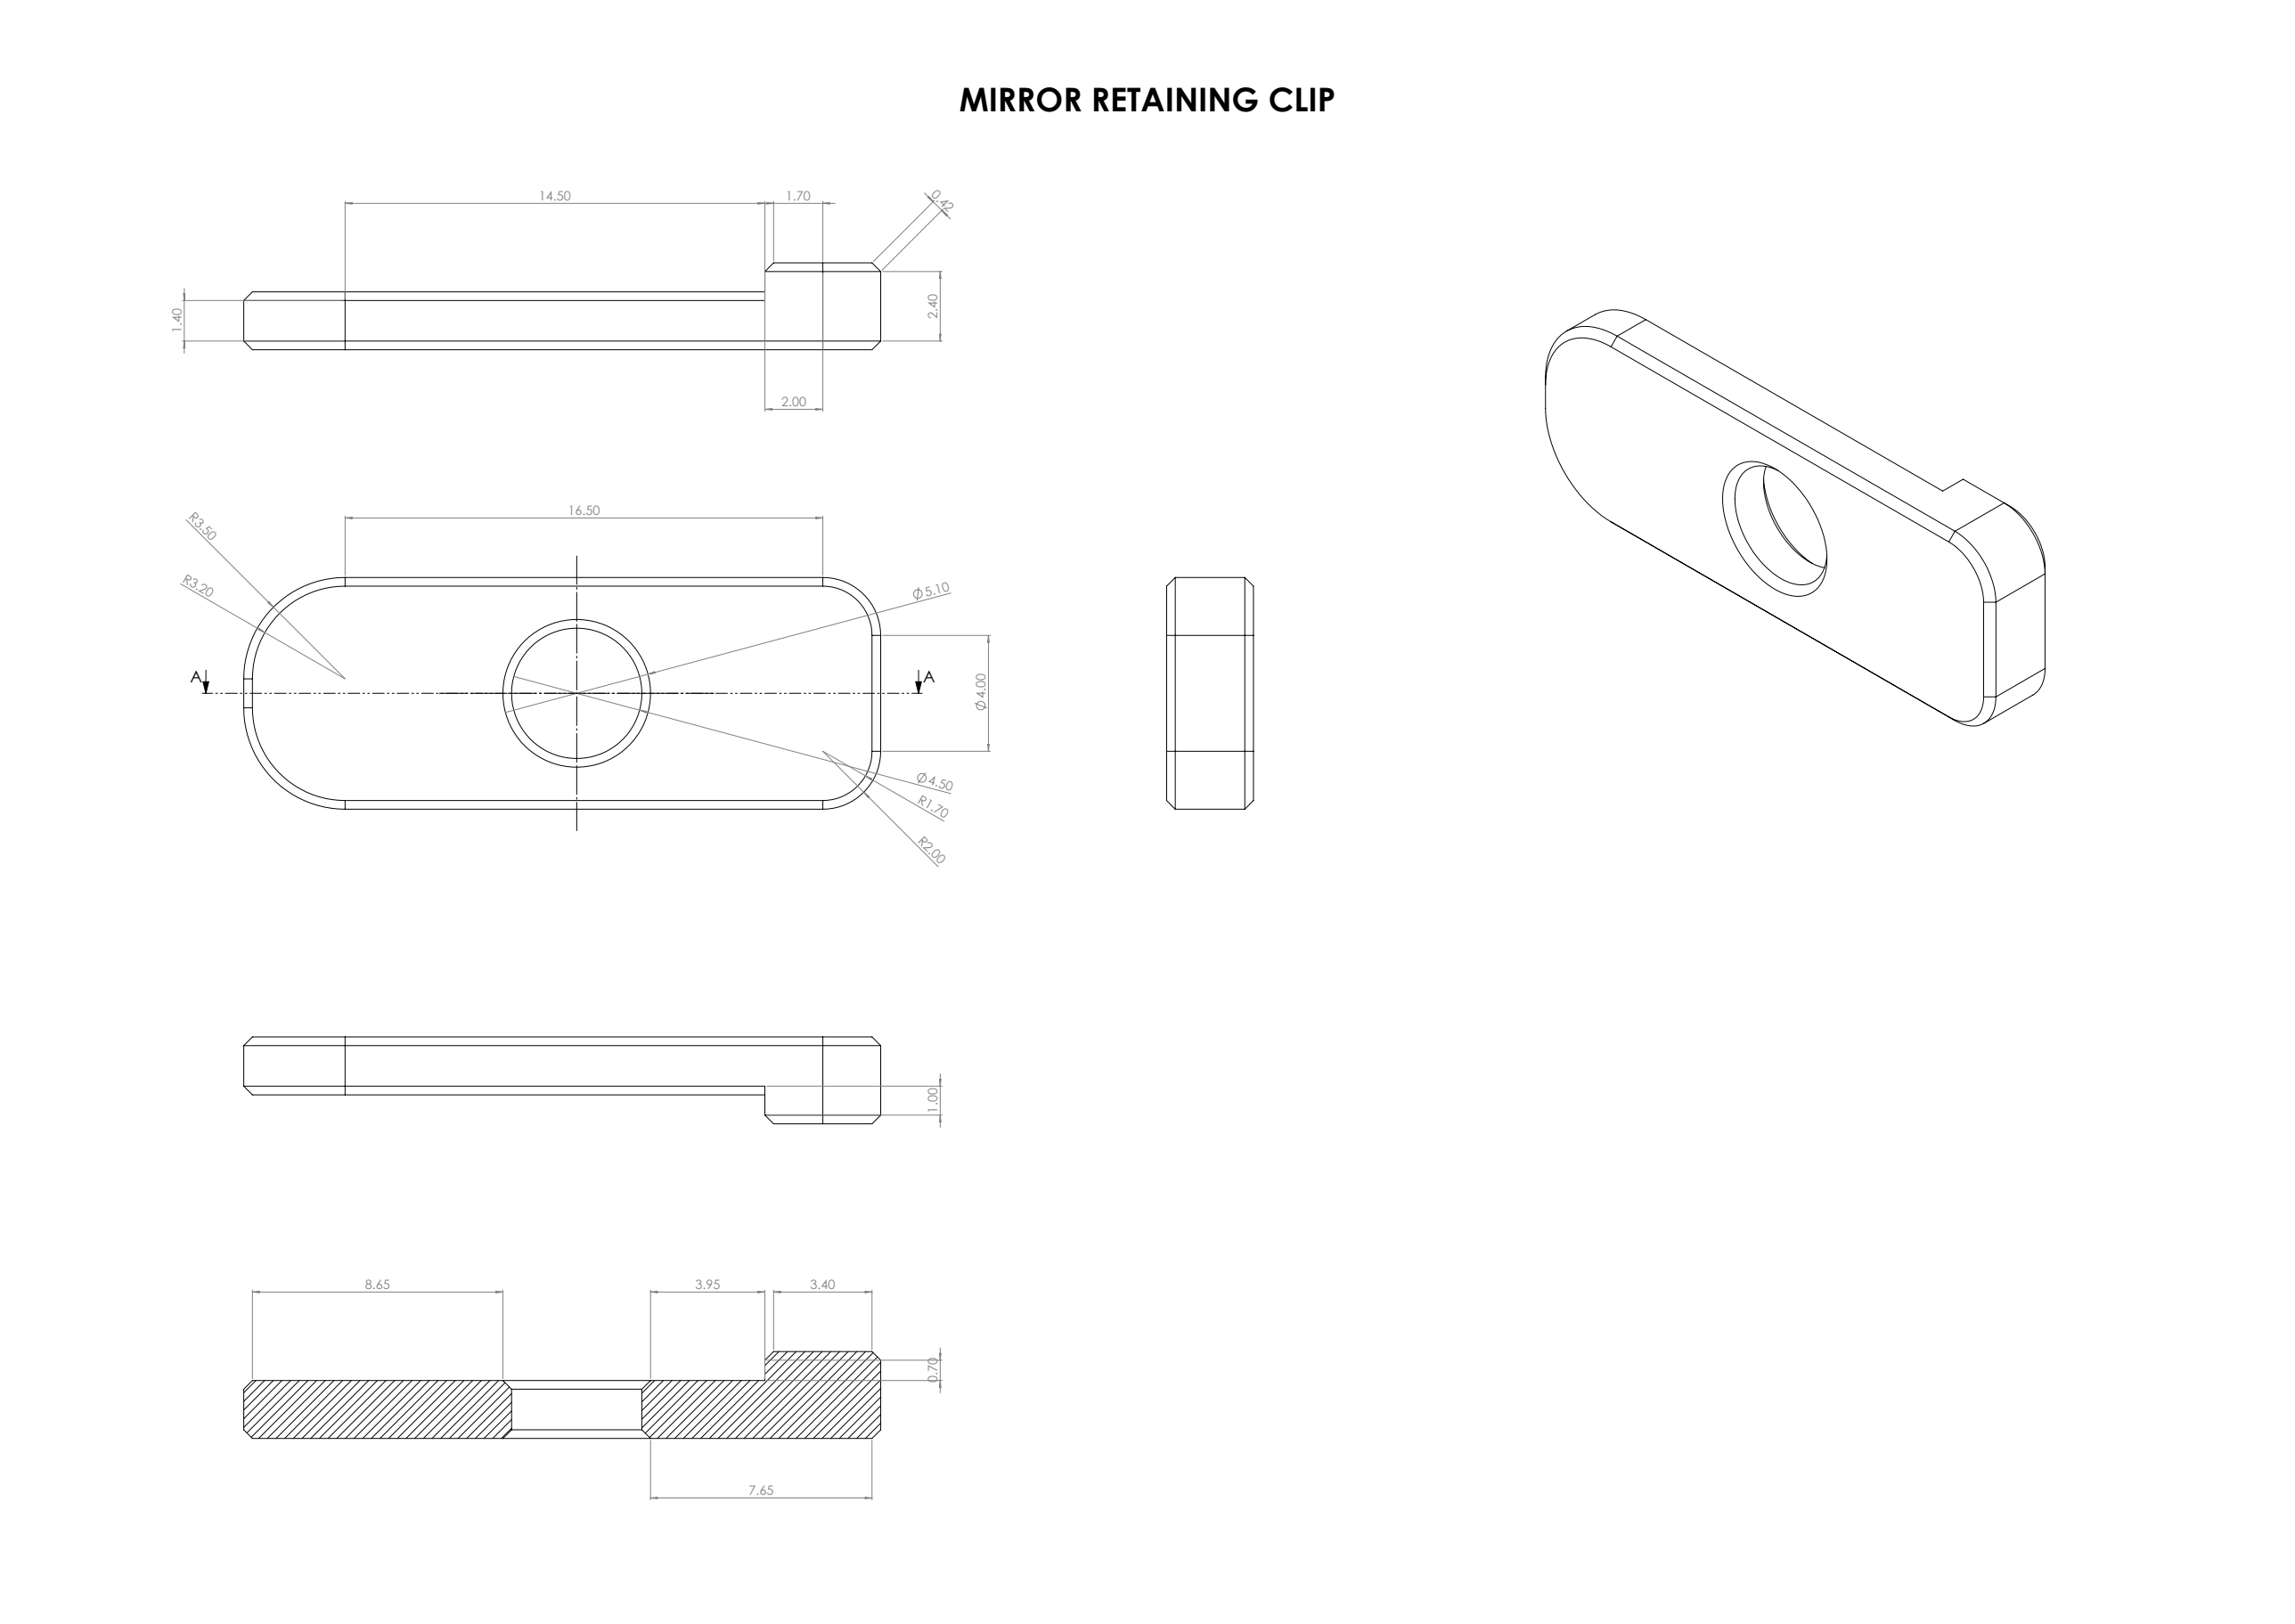
ISO-10303-21;
HEADER;
/* Generated by software containing ST-Developer
 * from STEP Tools, Inc. (www.steptools.com) 
 */

FILE_DESCRIPTION(
/* description */ (''),
/* implementation_level */ '2;1');

FILE_NAME(
/* name */ '09_Mirror_Retaining_Clip.step',
/* time_stamp */ '2026-10-19T22:59:19-07:00',
/* author */ (''),
/* organization */ (''),
/* preprocessor_version */ 'ST-DEVELOPER v20.2',
/* originating_system */ 'Autodesk Translation Framework v15.15.0.0',
/* authorisation */ '');

FILE_SCHEMA (('AUTOMOTIVE_DESIGN { 1 0 10303 214 3 1 1 }'));
ENDSEC;

DATA;
#10=MECHANICAL_DESIGN_GEOMETRIC_PRESENTATION_REPRESENTATION('',(#921),#53650);
#889=SHAPE_REPRESENTATION_RELATIONSHIP('SRR','None',#53734,#905);
#905=ADVANCED_BREP_SHAPE_REPRESENTATION('',(#937),#53644);
#921=STYLED_ITEM('',(#53951),#937);
#937=MANIFOLD_SOLID_BREP('Clip',#23313);
#1046=CYLINDRICAL_SURFACE('',#24534,0.225000000000001);
#1047=CYLINDRICAL_SURFACE('',#24564,0.2);
#1048=CYLINDRICAL_SURFACE('',#24581,0.2);
#1049=CYLINDRICAL_SURFACE('',#24583,0.35);
#1050=CYLINDRICAL_SURFACE('',#24585,0.35);
#1412=FACE_BOUND('',#4284,.T.);
#1413=FACE_BOUND('',#4287,.T.);
#1757=PLANE('',#24537);
#1758=PLANE('',#24542);
#1759=PLANE('',#24547);
#1760=PLANE('',#24550);
#1761=PLANE('',#24553);
#1762=PLANE('',#24554);
#1763=PLANE('',#24555);
#1764=PLANE('',#24559);
#1765=PLANE('',#24563);
#1766=PLANE('',#24566);
#1767=PLANE('',#24567);
#1768=PLANE('',#24568);
#1769=PLANE('',#24571);
#1770=PLANE('',#24574);
#1771=PLANE('',#24577);
#1772=PLANE('',#24579);
#1773=PLANE('',#24580);
#1774=PLANE('',#24582);
#1775=PLANE('',#24584);
#2818=FACE_OUTER_BOUND('',#4281,.T.);
#2819=FACE_OUTER_BOUND('',#4282,.T.);
#2820=FACE_OUTER_BOUND('',#4283,.T.);
#2821=FACE_OUTER_BOUND('',#4285,.T.);
#2822=FACE_OUTER_BOUND('',#4286,.T.);
#2823=FACE_OUTER_BOUND('',#4288,.T.);
#2824=FACE_OUTER_BOUND('',#4289,.T.);
#2825=FACE_OUTER_BOUND('',#4290,.T.);
#2826=FACE_OUTER_BOUND('',#4291,.T.);
#2827=FACE_OUTER_BOUND('',#4292,.T.);
#2828=FACE_OUTER_BOUND('',#4293,.T.);
#2829=FACE_OUTER_BOUND('',#4294,.T.);
#2830=FACE_OUTER_BOUND('',#4295,.T.);
#2831=FACE_OUTER_BOUND('',#4296,.T.);
#2832=FACE_OUTER_BOUND('',#4297,.T.);
#2833=FACE_OUTER_BOUND('',#4298,.T.);
#2834=FACE_OUTER_BOUND('',#4299,.T.);
#2835=FACE_OUTER_BOUND('',#4300,.T.);
#2836=FACE_OUTER_BOUND('',#4301,.T.);
#2837=FACE_OUTER_BOUND('',#4302,.T.);
#2838=FACE_OUTER_BOUND('',#4303,.T.);
#2839=FACE_OUTER_BOUND('',#4304,.T.);
#2840=FACE_OUTER_BOUND('',#4305,.T.);
#2841=FACE_OUTER_BOUND('',#4306,.T.);
#2842=FACE_OUTER_BOUND('',#4307,.T.);
#2843=FACE_OUTER_BOUND('',#4308,.T.);
#2844=FACE_OUTER_BOUND('',#4309,.T.);
#2845=FACE_OUTER_BOUND('',#4310,.T.);
#2846=FACE_OUTER_BOUND('',#4311,.T.);
#2847=FACE_OUTER_BOUND('',#4312,.T.);
#2848=FACE_OUTER_BOUND('',#4313,.T.);
#2849=FACE_OUTER_BOUND('',#4314,.T.);
#2850=FACE_OUTER_BOUND('',#4315,.T.);
#2851=FACE_OUTER_BOUND('',#4316,.T.);
#4281=EDGE_LOOP('',(#17627,#17628,#17629,#17630));
#4282=EDGE_LOOP('',(#17631,#17632,#17633,#17634,#17635));
#4283=EDGE_LOOP('',(#17636,#17637,#17638,#17639,#17640,#17641));
#4284=EDGE_LOOP('',(#17642));
#4285=EDGE_LOOP('',(#17643,#17644,#17645,#17646,#17647));
#4286=EDGE_LOOP('',(#17648,#17649,#17650,#17651,#17652,#17653,#17654,#17655));
#4287=EDGE_LOOP('',(#17656));
#4288=EDGE_LOOP('',(#17657,#17658,#17659,#17660));
#4289=EDGE_LOOP('',(#17661,#17662,#17663,#17664));
#4290=EDGE_LOOP('',(#17665,#17666,#17667,#17668));
#4291=EDGE_LOOP('',(#17669,#17670,#17671,#17672));
#4292=EDGE_LOOP('',(#17673,#17674,#17675,#17676));
#4293=EDGE_LOOP('',(#17677,#17678,#17679,#17680));
#4294=EDGE_LOOP('',(#17681,#17682,#17683,#17684));
#4295=EDGE_LOOP('',(#17685,#17686,#17687,#17688));
#4296=EDGE_LOOP('',(#17689,#17690,#17691,#17692));
#4297=EDGE_LOOP('',(#17693,#17694,#17695,#17696));
#4298=EDGE_LOOP('',(#17697,#17698,#17699,#17700));
#4299=EDGE_LOOP('',(#17701,#17702,#17703,#17704));
#4300=EDGE_LOOP('',(#17705,#17706,#17707,#17708,#17709,#17710));
#4301=EDGE_LOOP('',(#17711,#17712,#17713,#17714,#17715,#17716));
#4302=EDGE_LOOP('',(#17717,#17718,#17719,#17720,#17721,#17722));
#4303=EDGE_LOOP('',(#17723,#17724,#17725,#17726));
#4304=EDGE_LOOP('',(#17727,#17728,#17729,#17730));
#4305=EDGE_LOOP('',(#17731,#17732,#17733,#17734));
#4306=EDGE_LOOP('',(#17735,#17736,#17737,#17738));
#4307=EDGE_LOOP('',(#17739,#17740,#17741,#17742));
#4308=EDGE_LOOP('',(#17743,#17744,#17745,#17746));
#4309=EDGE_LOOP('',(#17747,#17748,#17749,#17750));
#4310=EDGE_LOOP('',(#17751,#17752,#17753,#17754));
#4311=EDGE_LOOP('',(#17755,#17756,#17757,#17758));
#4312=EDGE_LOOP('',(#17759,#17760,#17761,#17762));
#4313=EDGE_LOOP('',(#17763,#17764,#17765,#17766,#17767,#17768));
#4314=EDGE_LOOP('',(#17769,#17770,#17771,#17772));
#4315=EDGE_LOOP('',(#17773,#17774,#17775,#17776));
#4316=EDGE_LOOP('',(#17777,#17778,#17779,#17780));
#5506=CIRCLE('',#24532,0.255000000000001);
#5507=CIRCLE('',#24533,0.225000000000001);
#5508=CIRCLE('',#24535,0.225000000000001);
#5509=CIRCLE('',#24536,0.225000000000001);
#5510=CIRCLE('',#24538,0.32);
#5511=CIRCLE('',#24539,0.32);
#5512=CIRCLE('',#24541,0.255000000000001);
#5513=CIRCLE('',#24543,0.17);
#5514=CIRCLE('',#24544,0.17);
#5515=CIRCLE('',#24545,0.32);
#5516=CIRCLE('',#24546,0.32);
#5517=CIRCLE('',#24549,0.35);
#5518=CIRCLE('',#24552,0.35);
#5519=CIRCLE('',#24557,0.2);
#5520=CIRCLE('',#24558,0.17);
#5521=CIRCLE('',#24561,0.2);
#5522=CIRCLE('',#24562,0.17);
#5523=CIRCLE('',#24565,0.2);
#5524=CIRCLE('',#24570,0.2);
#5525=CIRCLE('',#24573,0.35);
#5526=CIRCLE('',#24576,0.35);
#6638=LINE('',#35987,#8483);
#6639=LINE('',#35991,#8484);
#6640=LINE('',#35998,#8485);
#6641=LINE('',#36002,#8486);
#6642=LINE('',#36006,#8487);
#6643=LINE('',#36007,#8488);
#6644=LINE('',#36011,#8489);
#6645=LINE('',#36017,#8490);
#6646=LINE('',#36021,#8491);
#6647=LINE('',#36025,#8492);
#6648=LINE('',#36028,#8493);
#6649=LINE('',#36031,#8494);
#6650=LINE('',#36033,#8495);
#6651=LINE('',#36034,#8496);
#6652=LINE('',#36037,#8497);
#6653=LINE('',#36041,#8498);
#6654=LINE('',#36042,#8499);
#6655=LINE('',#36045,#8500);
#6656=LINE('',#36049,#8501);
#6657=LINE('',#36050,#8502);
#6658=LINE('',#36054,#8503);
#6659=LINE('',#36056,#8504);
#6660=LINE('',#36058,#8505);
#6661=LINE('',#36059,#8506);
#6662=LINE('',#36062,#8507);
#6663=LINE('',#36064,#8508);
#6664=LINE('',#36065,#8509);
#6665=LINE('',#36069,#8510);
#6666=LINE('',#36075,#8511);
#6667=LINE('',#36076,#8512);
#6668=LINE('',#36077,#8513);
#6669=LINE('',#36081,#8514);
#6670=LINE('',#36085,#8515);
#6671=LINE('',#36086,#8516);
#6672=LINE('',#36089,#8517);
#6673=LINE('',#36092,#8518);
#6674=LINE('',#36095,#8519);
#6675=LINE('',#36096,#8520);
#6676=LINE('',#36097,#8521);
#6677=LINE('',#36099,#8522);
#6678=LINE('',#36103,#8523);
#6679=LINE('',#36106,#8524);
#6680=LINE('',#36109,#8525);
#6681=LINE('',#36110,#8526);
#6682=LINE('',#36113,#8527);
#6683=LINE('',#36117,#8528);
#6684=LINE('',#36118,#8529);
#6685=LINE('',#36120,#8530);
#6686=LINE('',#36123,#8531);
#6687=LINE('',#36125,#8532);
#6688=LINE('',#36127,#8533);
#6689=LINE('',#36129,#8534);
#6690=LINE('',#36131,#8535);
#6691=LINE('',#36133,#8536);
#6692=LINE('',#36135,#8537);
#6693=LINE('',#36137,#8538);
#8483=VECTOR('',#28514,0.240000000000001);
#8484=VECTOR('',#28519,0.225000000000001);
#8485=VECTOR('',#28526,1.);
#8486=VECTOR('',#28529,1.);
#8487=VECTOR('',#28532,1.);
#8488=VECTOR('',#28533,1.);
#8489=VECTOR('',#28538,0.240000000000001);
#8490=VECTOR('',#28543,1.);
#8491=VECTOR('',#28546,1.);
#8492=VECTOR('',#28549,1.);
#8493=VECTOR('',#28552,1.);
#8494=VECTOR('',#28555,1.);
#8495=VECTOR('',#28556,1.);
#8496=VECTOR('',#28557,1.);
#8497=VECTOR('',#28560,1.);
#8498=VECTOR('',#28565,1.);
#8499=VECTOR('',#28566,1.);
#8500=VECTOR('',#28569,1.);
#8501=VECTOR('',#28574,1.);
#8502=VECTOR('',#28575,1.);
#8503=VECTOR('',#28578,1.);
#8504=VECTOR('',#28579,1.);
#8505=VECTOR('',#28580,1.);
#8506=VECTOR('',#28581,1.);
#8507=VECTOR('',#28584,1.);
#8508=VECTOR('',#28585,1.);
#8509=VECTOR('',#28586,1.);
#8510=VECTOR('',#28589,1.);
#8511=VECTOR('',#28596,1.);
#8512=VECTOR('',#28597,1.);
#8513=VECTOR('',#28598,1.);
#8514=VECTOR('',#28601,1.);
#8515=VECTOR('',#28608,1.);
#8516=VECTOR('',#28609,1.);
#8517=VECTOR('',#28612,1.);
#8518=VECTOR('',#28615,1.);
#8519=VECTOR('',#28618,1.);
#8520=VECTOR('',#28619,1.);
#8521=VECTOR('',#28620,1.);
#8522=VECTOR('',#28623,1.);
#8523=VECTOR('',#28628,1.);
#8524=VECTOR('',#28631,1.);
#8525=VECTOR('',#28634,1.);
#8526=VECTOR('',#28635,1.);
#8527=VECTOR('',#28638,1.);
#8528=VECTOR('',#28643,1.);
#8529=VECTOR('',#28644,1.);
#8530=VECTOR('',#28647,1.);
#8531=VECTOR('',#28652,1.);
#8532=VECTOR('',#28655,1.);
#8533=VECTOR('',#28658,1.);
#8534=VECTOR('',#28661,1.);
#8535=VECTOR('',#28664,1.);
#8536=VECTOR('',#28667,1.);
#8537=VECTOR('',#28670,1.);
#8538=VECTOR('',#28673,1.);
#10337=VERTEX_POINT('',#35984);
#10338=VERTEX_POINT('',#35986);
#10339=VERTEX_POINT('',#35990);
#10340=VERTEX_POINT('',#35992);
#10341=VERTEX_POINT('',#35996);
#10342=VERTEX_POINT('',#35997);
#10343=VERTEX_POINT('',#35999);
#10344=VERTEX_POINT('',#36001);
#10345=VERTEX_POINT('',#36003);
#10346=VERTEX_POINT('',#36005);
#10347=VERTEX_POINT('',#36009);
#10348=VERTEX_POINT('',#36013);
#10349=VERTEX_POINT('',#36014);
#10350=VERTEX_POINT('',#36016);
#10351=VERTEX_POINT('',#36018);
#10352=VERTEX_POINT('',#36020);
#10353=VERTEX_POINT('',#36022);
#10354=VERTEX_POINT('',#36024);
#10355=VERTEX_POINT('',#36026);
#10356=VERTEX_POINT('',#36030);
#10357=VERTEX_POINT('',#36032);
#10358=VERTEX_POINT('',#36036);
#10359=VERTEX_POINT('',#36040);
#10360=VERTEX_POINT('',#36044);
#10361=VERTEX_POINT('',#36048);
#10362=VERTEX_POINT('',#36052);
#10363=VERTEX_POINT('',#36053);
#10364=VERTEX_POINT('',#36055);
#10365=VERTEX_POINT('',#36057);
#10366=VERTEX_POINT('',#36061);
#10367=VERTEX_POINT('',#36063);
#10368=VERTEX_POINT('',#36067);
#10369=VERTEX_POINT('',#36068);
#10370=VERTEX_POINT('',#36073);
#10371=VERTEX_POINT('',#36074);
#10372=VERTEX_POINT('',#36079);
#10373=VERTEX_POINT('',#36080);
#10374=VERTEX_POINT('',#36088);
#10375=VERTEX_POINT('',#36090);
#10376=VERTEX_POINT('',#36094);
#10377=VERTEX_POINT('',#36102);
#10378=VERTEX_POINT('',#36104);
#10379=VERTEX_POINT('',#36108);
#10380=VERTEX_POINT('',#36112);
#10381=VERTEX_POINT('',#36116);
#12991=EDGE_CURVE('',#10337,#10337,#5506,.T.);
#12992=EDGE_CURVE('',#10337,#10338,#6638,.T.);
#12993=EDGE_CURVE('',#10338,#10338,#5507,.T.);
#12994=EDGE_CURVE('',#10338,#10339,#6639,.T.);
#12995=EDGE_CURVE('',#10340,#10339,#5508,.T.);
#12996=EDGE_CURVE('',#10339,#10340,#5509,.T.);
#12997=EDGE_CURVE('',#10341,#10342,#6640,.T.);
#12998=EDGE_CURVE('',#10343,#10341,#5510,.T.);
#12999=EDGE_CURVE('',#10344,#10343,#6641,.T.);
#13000=EDGE_CURVE('',#10345,#10344,#5511,.T.);
#13001=EDGE_CURVE('',#10346,#10345,#6642,.T.);
#13002=EDGE_CURVE('',#10346,#10342,#6643,.T.);
#13003=EDGE_CURVE('',#10347,#10347,#5512,.T.);
#13004=EDGE_CURVE('',#10347,#10340,#6644,.T.);
#13005=EDGE_CURVE('',#10348,#10349,#5513,.T.);
#13006=EDGE_CURVE('',#10350,#10348,#6645,.T.);
#13007=EDGE_CURVE('',#10351,#10350,#5514,.T.);
#13008=EDGE_CURVE('',#10352,#10351,#6646,.T.);
#13009=EDGE_CURVE('',#10353,#10352,#5515,.T.);
#13010=EDGE_CURVE('',#10354,#10353,#6647,.T.);
#13011=EDGE_CURVE('',#10355,#10354,#5516,.T.);
#13012=EDGE_CURVE('',#10349,#10355,#6648,.T.);
#13013=EDGE_CURVE('',#10356,#10346,#6649,.F.);
#13014=EDGE_CURVE('',#10345,#10357,#6650,.T.);
#13015=EDGE_CURVE('',#10357,#10356,#6651,.T.);
#13016=EDGE_CURVE('',#10344,#10358,#6652,.T.);
#13017=EDGE_CURVE('',#10358,#10357,#5517,.T.);
#13018=EDGE_CURVE('',#10343,#10359,#6653,.T.);
#13019=EDGE_CURVE('',#10359,#10358,#6654,.T.);
#13020=EDGE_CURVE('',#10341,#10360,#6655,.T.);
#13021=EDGE_CURVE('',#10360,#10359,#5518,.T.);
#13022=EDGE_CURVE('',#10342,#10361,#6656,.F.);
#13023=EDGE_CURVE('',#10361,#10360,#6657,.T.);
#13024=EDGE_CURVE('',#10362,#10363,#6658,.T.);
#13025=EDGE_CURVE('',#10363,#10364,#6659,.T.);
#13026=EDGE_CURVE('',#10364,#10365,#6660,.T.);
#13027=EDGE_CURVE('',#10365,#10362,#6661,.T.);
#13028=EDGE_CURVE('',#10365,#10366,#6662,.T.);
#13029=EDGE_CURVE('',#10366,#10367,#6663,.T.);
#13030=EDGE_CURVE('',#10367,#10362,#6664,.T.);
#13031=EDGE_CURVE('',#10368,#10369,#6665,.T.);
#13032=EDGE_CURVE('',#10369,#10367,#5519,.T.);
#13033=EDGE_CURVE('',#10366,#10368,#5520,.T.);
#13034=EDGE_CURVE('',#10370,#10371,#6666,.T.);
#13035=EDGE_CURVE('',#10371,#10369,#6667,.T.);
#13036=EDGE_CURVE('',#10368,#10370,#6668,.T.);
#13037=EDGE_CURVE('',#10372,#10373,#6669,.T.);
#13038=EDGE_CURVE('',#10373,#10371,#5521,.T.);
#13039=EDGE_CURVE('',#10370,#10372,#5522,.T.);
#13040=EDGE_CURVE('',#10363,#10373,#6670,.T.);
#13041=EDGE_CURVE('',#10372,#10364,#6671,.T.);
#13042=EDGE_CURVE('',#10373,#10374,#6672,.T.);
#13043=EDGE_CURVE('',#10375,#10374,#5523,.T.);
#13044=EDGE_CURVE('',#10375,#10371,#6673,.T.);
#13045=EDGE_CURVE('',#10376,#10357,#6674,.T.);
#13046=EDGE_CURVE('',#10374,#10376,#6675,.T.);
#13047=EDGE_CURVE('',#10363,#10356,#6676,.T.);
#13048=EDGE_CURVE('',#10362,#10361,#6677,.T.);
#13049=EDGE_CURVE('',#10349,#10377,#6678,.T.);
#13050=EDGE_CURVE('',#10377,#10378,#5524,.T.);
#13051=EDGE_CURVE('',#10378,#10348,#6679,.T.);
#13052=EDGE_CURVE('',#10355,#10379,#6680,.T.);
#13053=EDGE_CURVE('',#10379,#10377,#6681,.T.);
#13054=EDGE_CURVE('',#10354,#10380,#6682,.T.);
#13055=EDGE_CURVE('',#10380,#10379,#5525,.T.);
#13056=EDGE_CURVE('',#10353,#10381,#6683,.T.);
#13057=EDGE_CURVE('',#10381,#10380,#6684,.T.);
#13058=EDGE_CURVE('',#10352,#10376,#6685,.T.);
#13059=EDGE_CURVE('',#10376,#10381,#5526,.T.);
#13060=EDGE_CURVE('',#10351,#10374,#6686,.T.);
#13061=EDGE_CURVE('',#10350,#10375,#6687,.T.);
#13062=EDGE_CURVE('',#10378,#10375,#6688,.T.);
#13063=EDGE_CURVE('',#10369,#10378,#6689,.T.);
#13064=EDGE_CURVE('',#10377,#10367,#6690,.T.);
#13065=EDGE_CURVE('',#10360,#10379,#6691,.T.);
#13066=EDGE_CURVE('',#10380,#10359,#6692,.T.);
#13067=EDGE_CURVE('',#10358,#10381,#6693,.T.);
#17627=ORIENTED_EDGE('',*,*,#12991,.T.);
#17628=ORIENTED_EDGE('',*,*,#12992,.T.);
#17629=ORIENTED_EDGE('',*,*,#12993,.T.);
#17630=ORIENTED_EDGE('',*,*,#12992,.F.);
#17631=ORIENTED_EDGE('',*,*,#12993,.F.);
#17632=ORIENTED_EDGE('',*,*,#12994,.T.);
#17633=ORIENTED_EDGE('',*,*,#12995,.F.);
#17634=ORIENTED_EDGE('',*,*,#12996,.F.);
#17635=ORIENTED_EDGE('',*,*,#12994,.F.);
#17636=ORIENTED_EDGE('',*,*,#12997,.F.);
#17637=ORIENTED_EDGE('',*,*,#12998,.F.);
#17638=ORIENTED_EDGE('',*,*,#12999,.F.);
#17639=ORIENTED_EDGE('',*,*,#13000,.F.);
#17640=ORIENTED_EDGE('',*,*,#13001,.F.);
#17641=ORIENTED_EDGE('',*,*,#13002,.T.);
#17642=ORIENTED_EDGE('',*,*,#12991,.F.);
#17643=ORIENTED_EDGE('',*,*,#13003,.T.);
#17644=ORIENTED_EDGE('',*,*,#13004,.T.);
#17645=ORIENTED_EDGE('',*,*,#12995,.T.);
#17646=ORIENTED_EDGE('',*,*,#12996,.T.);
#17647=ORIENTED_EDGE('',*,*,#13004,.F.);
#17648=ORIENTED_EDGE('',*,*,#13005,.F.);
#17649=ORIENTED_EDGE('',*,*,#13006,.F.);
#17650=ORIENTED_EDGE('',*,*,#13007,.F.);
#17651=ORIENTED_EDGE('',*,*,#13008,.F.);
#17652=ORIENTED_EDGE('',*,*,#13009,.F.);
#17653=ORIENTED_EDGE('',*,*,#13010,.F.);
#17654=ORIENTED_EDGE('',*,*,#13011,.F.);
#17655=ORIENTED_EDGE('',*,*,#13012,.F.);
#17656=ORIENTED_EDGE('',*,*,#13003,.F.);
#17657=ORIENTED_EDGE('',*,*,#13013,.T.);
#17658=ORIENTED_EDGE('',*,*,#13001,.T.);
#17659=ORIENTED_EDGE('',*,*,#13014,.T.);
#17660=ORIENTED_EDGE('',*,*,#13015,.T.);
#17661=ORIENTED_EDGE('',*,*,#13016,.T.);
#17662=ORIENTED_EDGE('',*,*,#13017,.T.);
#17663=ORIENTED_EDGE('',*,*,#13014,.F.);
#17664=ORIENTED_EDGE('',*,*,#13000,.T.);
#17665=ORIENTED_EDGE('',*,*,#13018,.T.);
#17666=ORIENTED_EDGE('',*,*,#13019,.T.);
#17667=ORIENTED_EDGE('',*,*,#13016,.F.);
#17668=ORIENTED_EDGE('',*,*,#12999,.T.);
#17669=ORIENTED_EDGE('',*,*,#13020,.T.);
#17670=ORIENTED_EDGE('',*,*,#13021,.T.);
#17671=ORIENTED_EDGE('',*,*,#13018,.F.);
#17672=ORIENTED_EDGE('',*,*,#12998,.T.);
#17673=ORIENTED_EDGE('',*,*,#13022,.T.);
#17674=ORIENTED_EDGE('',*,*,#13023,.T.);
#17675=ORIENTED_EDGE('',*,*,#13020,.F.);
#17676=ORIENTED_EDGE('',*,*,#12997,.T.);
#17677=ORIENTED_EDGE('',*,*,#13024,.T.);
#17678=ORIENTED_EDGE('',*,*,#13025,.T.);
#17679=ORIENTED_EDGE('',*,*,#13026,.T.);
#17680=ORIENTED_EDGE('',*,*,#13027,.T.);
#17681=ORIENTED_EDGE('',*,*,#13028,.T.);
#17682=ORIENTED_EDGE('',*,*,#13029,.T.);
#17683=ORIENTED_EDGE('',*,*,#13030,.T.);
#17684=ORIENTED_EDGE('',*,*,#13027,.F.);
#17685=ORIENTED_EDGE('',*,*,#13031,.T.);
#17686=ORIENTED_EDGE('',*,*,#13032,.T.);
#17687=ORIENTED_EDGE('',*,*,#13029,.F.);
#17688=ORIENTED_EDGE('',*,*,#13033,.T.);
#17689=ORIENTED_EDGE('',*,*,#13034,.T.);
#17690=ORIENTED_EDGE('',*,*,#13035,.T.);
#17691=ORIENTED_EDGE('',*,*,#13031,.F.);
#17692=ORIENTED_EDGE('',*,*,#13036,.T.);
#17693=ORIENTED_EDGE('',*,*,#13037,.T.);
#17694=ORIENTED_EDGE('',*,*,#13038,.T.);
#17695=ORIENTED_EDGE('',*,*,#13034,.F.);
#17696=ORIENTED_EDGE('',*,*,#13039,.T.);
#17697=ORIENTED_EDGE('',*,*,#13040,.T.);
#17698=ORIENTED_EDGE('',*,*,#13037,.F.);
#17699=ORIENTED_EDGE('',*,*,#13041,.T.);
#17700=ORIENTED_EDGE('',*,*,#13025,.F.);
#17701=ORIENTED_EDGE('',*,*,#13038,.F.);
#17702=ORIENTED_EDGE('',*,*,#13042,.T.);
#17703=ORIENTED_EDGE('',*,*,#13043,.F.);
#17704=ORIENTED_EDGE('',*,*,#13044,.T.);
#17705=ORIENTED_EDGE('',*,*,#13015,.F.);
#17706=ORIENTED_EDGE('',*,*,#13045,.F.);
#17707=ORIENTED_EDGE('',*,*,#13046,.F.);
#17708=ORIENTED_EDGE('',*,*,#13042,.F.);
#17709=ORIENTED_EDGE('',*,*,#13040,.F.);
#17710=ORIENTED_EDGE('',*,*,#13047,.T.);
#17711=ORIENTED_EDGE('',*,*,#13024,.F.);
#17712=ORIENTED_EDGE('',*,*,#13048,.T.);
#17713=ORIENTED_EDGE('',*,*,#13022,.F.);
#17714=ORIENTED_EDGE('',*,*,#13002,.F.);
#17715=ORIENTED_EDGE('',*,*,#13013,.F.);
#17716=ORIENTED_EDGE('',*,*,#13047,.F.);
#17717=ORIENTED_EDGE('',*,*,#13026,.F.);
#17718=ORIENTED_EDGE('',*,*,#13041,.F.);
#17719=ORIENTED_EDGE('',*,*,#13039,.F.);
#17720=ORIENTED_EDGE('',*,*,#13036,.F.);
#17721=ORIENTED_EDGE('',*,*,#13033,.F.);
#17722=ORIENTED_EDGE('',*,*,#13028,.F.);
#17723=ORIENTED_EDGE('',*,*,#13049,.T.);
#17724=ORIENTED_EDGE('',*,*,#13050,.T.);
#17725=ORIENTED_EDGE('',*,*,#13051,.T.);
#17726=ORIENTED_EDGE('',*,*,#13005,.T.);
#17727=ORIENTED_EDGE('',*,*,#13049,.F.);
#17728=ORIENTED_EDGE('',*,*,#13012,.T.);
#17729=ORIENTED_EDGE('',*,*,#13052,.T.);
#17730=ORIENTED_EDGE('',*,*,#13053,.T.);
#17731=ORIENTED_EDGE('',*,*,#13054,.T.);
#17732=ORIENTED_EDGE('',*,*,#13055,.T.);
#17733=ORIENTED_EDGE('',*,*,#13052,.F.);
#17734=ORIENTED_EDGE('',*,*,#13011,.T.);
#17735=ORIENTED_EDGE('',*,*,#13054,.F.);
#17736=ORIENTED_EDGE('',*,*,#13010,.T.);
#17737=ORIENTED_EDGE('',*,*,#13056,.T.);
#17738=ORIENTED_EDGE('',*,*,#13057,.T.);
#17739=ORIENTED_EDGE('',*,*,#13058,.T.);
#17740=ORIENTED_EDGE('',*,*,#13059,.T.);
#17741=ORIENTED_EDGE('',*,*,#13056,.F.);
#17742=ORIENTED_EDGE('',*,*,#13009,.T.);
#17743=ORIENTED_EDGE('',*,*,#13058,.F.);
#17744=ORIENTED_EDGE('',*,*,#13008,.T.);
#17745=ORIENTED_EDGE('',*,*,#13060,.T.);
#17746=ORIENTED_EDGE('',*,*,#13046,.T.);
#17747=ORIENTED_EDGE('',*,*,#13061,.T.);
#17748=ORIENTED_EDGE('',*,*,#13043,.T.);
#17749=ORIENTED_EDGE('',*,*,#13060,.F.);
#17750=ORIENTED_EDGE('',*,*,#13007,.T.);
#17751=ORIENTED_EDGE('',*,*,#13061,.F.);
#17752=ORIENTED_EDGE('',*,*,#13006,.T.);
#17753=ORIENTED_EDGE('',*,*,#13051,.F.);
#17754=ORIENTED_EDGE('',*,*,#13062,.T.);
#17755=ORIENTED_EDGE('',*,*,#13035,.F.);
#17756=ORIENTED_EDGE('',*,*,#13044,.F.);
#17757=ORIENTED_EDGE('',*,*,#13062,.F.);
#17758=ORIENTED_EDGE('',*,*,#13063,.F.);
#17759=ORIENTED_EDGE('',*,*,#13032,.F.);
#17760=ORIENTED_EDGE('',*,*,#13063,.T.);
#17761=ORIENTED_EDGE('',*,*,#13050,.F.);
#17762=ORIENTED_EDGE('',*,*,#13064,.T.);
#17763=ORIENTED_EDGE('',*,*,#13048,.F.);
#17764=ORIENTED_EDGE('',*,*,#13030,.F.);
#17765=ORIENTED_EDGE('',*,*,#13064,.F.);
#17766=ORIENTED_EDGE('',*,*,#13053,.F.);
#17767=ORIENTED_EDGE('',*,*,#13065,.F.);
#17768=ORIENTED_EDGE('',*,*,#13023,.F.);
#17769=ORIENTED_EDGE('',*,*,#13021,.F.);
#17770=ORIENTED_EDGE('',*,*,#13065,.T.);
#17771=ORIENTED_EDGE('',*,*,#13055,.F.);
#17772=ORIENTED_EDGE('',*,*,#13066,.T.);
#17773=ORIENTED_EDGE('',*,*,#13019,.F.);
#17774=ORIENTED_EDGE('',*,*,#13066,.F.);
#17775=ORIENTED_EDGE('',*,*,#13057,.F.);
#17776=ORIENTED_EDGE('',*,*,#13067,.F.);
#17777=ORIENTED_EDGE('',*,*,#13017,.F.);
#17778=ORIENTED_EDGE('',*,*,#13067,.T.);
#17779=ORIENTED_EDGE('',*,*,#13059,.F.);
#17780=ORIENTED_EDGE('',*,*,#13045,.T.);
#21947=CONICAL_SURFACE('',#24531,0.240000000000001,0.785398163397452);
#21948=CONICAL_SURFACE('',#24540,0.240000000000001,0.785398163397452);
#21949=CONICAL_SURFACE('',#24548,0.335,0.785398163397444);
#21950=CONICAL_SURFACE('',#24551,0.335,0.785398163397446);
#21951=CONICAL_SURFACE('',#24556,0.185,0.785398163397452);
#21952=CONICAL_SURFACE('',#24560,0.185,0.785398163397455);
#21953=CONICAL_SURFACE('',#24569,0.185,0.785398163397451);
#21954=CONICAL_SURFACE('',#24572,0.335,0.785398163397445);
#21955=CONICAL_SURFACE('',#24575,0.335,0.785398163397444);
#21956=CONICAL_SURFACE('',#24578,0.185,0.785398163397455);
#22557=ADVANCED_FACE('',(#2818),#21947,.F.);
#22558=ADVANCED_FACE('',(#2819),#1046,.F.);
#22559=ADVANCED_FACE('',(#2820,#1412),#1757,.F.);
#22560=ADVANCED_FACE('',(#2821),#21948,.F.);
#22561=ADVANCED_FACE('',(#2822,#1413),#1758,.T.);
#22562=ADVANCED_FACE('',(#2823),#1759,.T.);
#22563=ADVANCED_FACE('',(#2824),#21949,.T.);
#22564=ADVANCED_FACE('',(#2825),#1760,.T.);
#22565=ADVANCED_FACE('',(#2826),#21950,.T.);
#22566=ADVANCED_FACE('',(#2827),#1761,.T.);
#22567=ADVANCED_FACE('',(#2828),#1762,.T.);
#22568=ADVANCED_FACE('',(#2829),#1763,.T.);
#22569=ADVANCED_FACE('',(#2830),#21951,.T.);
#22570=ADVANCED_FACE('',(#2831),#1764,.T.);
#22571=ADVANCED_FACE('',(#2832),#21952,.T.);
#22572=ADVANCED_FACE('',(#2833),#1765,.T.);
#22573=ADVANCED_FACE('',(#2834),#1047,.T.);
#22574=ADVANCED_FACE('',(#2835),#1766,.T.);
#22575=ADVANCED_FACE('',(#2836),#1767,.T.);
#22576=ADVANCED_FACE('',(#2837),#1768,.F.);
#22577=ADVANCED_FACE('',(#2838),#21953,.T.);
#22578=ADVANCED_FACE('',(#2839),#1769,.T.);
#22579=ADVANCED_FACE('',(#2840),#21954,.T.);
#22580=ADVANCED_FACE('',(#2841),#1770,.T.);
#22581=ADVANCED_FACE('',(#2842),#21955,.T.);
#22582=ADVANCED_FACE('',(#2843),#1771,.T.);
#22583=ADVANCED_FACE('',(#2844),#21956,.T.);
#22584=ADVANCED_FACE('',(#2845),#1772,.T.);
#22585=ADVANCED_FACE('',(#2846),#1773,.T.);
#22586=ADVANCED_FACE('',(#2847),#1048,.T.);
#22587=ADVANCED_FACE('',(#2848),#1774,.T.);
#22588=ADVANCED_FACE('',(#2849),#1049,.T.);
#22589=ADVANCED_FACE('',(#2850),#1775,.T.);
#22590=ADVANCED_FACE('',(#2851),#1050,.T.);
#23313=CLOSED_SHELL('',(#22557,#22558,#22559,#22560,#22561,#22562,#22563,
#22564,#22565,#22566,#22567,#22568,#22569,#22570,#22571,#22572,#22573,#22574,
#22575,#22576,#22577,#22578,#22579,#22580,#22581,#22582,#22583,#22584,#22585,
#22586,#22587,#22588,#22589,#22590));
#24530=AXIS2_PLACEMENT_3D('',#35982,#28508,#28509);
#24531=AXIS2_PLACEMENT_3D('',#35983,#28510,#28511);
#24532=AXIS2_PLACEMENT_3D('',#35985,#28512,#28513);
#24533=AXIS2_PLACEMENT_3D('',#35988,#28515,#28516);
#24534=AXIS2_PLACEMENT_3D('',#35989,#28517,#28518);
#24535=AXIS2_PLACEMENT_3D('',#35993,#28520,#28521);
#24536=AXIS2_PLACEMENT_3D('',#35994,#28522,#28523);
#24537=AXIS2_PLACEMENT_3D('',#35995,#28524,#28525);
#24538=AXIS2_PLACEMENT_3D('',#36000,#28527,#28528);
#24539=AXIS2_PLACEMENT_3D('',#36004,#28530,#28531);
#24540=AXIS2_PLACEMENT_3D('',#36008,#28534,#28535);
#24541=AXIS2_PLACEMENT_3D('',#36010,#28536,#28537);
#24542=AXIS2_PLACEMENT_3D('',#36012,#28539,#28540);
#24543=AXIS2_PLACEMENT_3D('',#36015,#28541,#28542);
#24544=AXIS2_PLACEMENT_3D('',#36019,#28544,#28545);
#24545=AXIS2_PLACEMENT_3D('',#36023,#28547,#28548);
#24546=AXIS2_PLACEMENT_3D('',#36027,#28550,#28551);
#24547=AXIS2_PLACEMENT_3D('',#36029,#28553,#28554);
#24548=AXIS2_PLACEMENT_3D('',#36035,#28558,#28559);
#24549=AXIS2_PLACEMENT_3D('',#36038,#28561,#28562);
#24550=AXIS2_PLACEMENT_3D('',#36039,#28563,#28564);
#24551=AXIS2_PLACEMENT_3D('',#36043,#28567,#28568);
#24552=AXIS2_PLACEMENT_3D('',#36046,#28570,#28571);
#24553=AXIS2_PLACEMENT_3D('',#36047,#28572,#28573);
#24554=AXIS2_PLACEMENT_3D('',#36051,#28576,#28577);
#24555=AXIS2_PLACEMENT_3D('',#36060,#28582,#28583);
#24556=AXIS2_PLACEMENT_3D('',#36066,#28587,#28588);
#24557=AXIS2_PLACEMENT_3D('',#36070,#28590,#28591);
#24558=AXIS2_PLACEMENT_3D('',#36071,#28592,#28593);
#24559=AXIS2_PLACEMENT_3D('',#36072,#28594,#28595);
#24560=AXIS2_PLACEMENT_3D('',#36078,#28599,#28600);
#24561=AXIS2_PLACEMENT_3D('',#36082,#28602,#28603);
#24562=AXIS2_PLACEMENT_3D('',#36083,#28604,#28605);
#24563=AXIS2_PLACEMENT_3D('',#36084,#28606,#28607);
#24564=AXIS2_PLACEMENT_3D('',#36087,#28610,#28611);
#24565=AXIS2_PLACEMENT_3D('',#36091,#28613,#28614);
#24566=AXIS2_PLACEMENT_3D('',#36093,#28616,#28617);
#24567=AXIS2_PLACEMENT_3D('',#36098,#28621,#28622);
#24568=AXIS2_PLACEMENT_3D('',#36100,#28624,#28625);
#24569=AXIS2_PLACEMENT_3D('',#36101,#28626,#28627);
#24570=AXIS2_PLACEMENT_3D('',#36105,#28629,#28630);
#24571=AXIS2_PLACEMENT_3D('',#36107,#28632,#28633);
#24572=AXIS2_PLACEMENT_3D('',#36111,#28636,#28637);
#24573=AXIS2_PLACEMENT_3D('',#36114,#28639,#28640);
#24574=AXIS2_PLACEMENT_3D('',#36115,#28641,#28642);
#24575=AXIS2_PLACEMENT_3D('',#36119,#28645,#28646);
#24576=AXIS2_PLACEMENT_3D('',#36121,#28648,#28649);
#24577=AXIS2_PLACEMENT_3D('',#36122,#28650,#28651);
#24578=AXIS2_PLACEMENT_3D('',#36124,#28653,#28654);
#24579=AXIS2_PLACEMENT_3D('',#36126,#28656,#28657);
#24580=AXIS2_PLACEMENT_3D('',#36128,#28659,#28660);
#24581=AXIS2_PLACEMENT_3D('',#36130,#28662,#28663);
#24582=AXIS2_PLACEMENT_3D('',#36132,#28665,#28666);
#24583=AXIS2_PLACEMENT_3D('',#36134,#28668,#28669);
#24584=AXIS2_PLACEMENT_3D('',#36136,#28671,#28672);
#24585=AXIS2_PLACEMENT_3D('',#36138,#28674,#28675);
#28508=DIRECTION('axis',(0.,0.,1.));
#28509=DIRECTION('refdir',(1.,0.,0.));
#28510=DIRECTION('center_axis',(0.,0.,-1.));
#28511=DIRECTION('ref_axis',(1.,0.,0.));
#28512=DIRECTION('center_axis',(0.,0.,-1.));
#28513=DIRECTION('ref_axis',(1.,0.,0.));
#28514=DIRECTION('',(0.70710678118655,-8.65956056235497E-17,0.707106781186545));
#28515=DIRECTION('center_axis',(0.,0.,1.));
#28516=DIRECTION('ref_axis',(1.,0.,0.));
#28517=DIRECTION('center_axis',(0.,0.,1.));
#28518=DIRECTION('ref_axis',(1.,0.,0.));
#28519=DIRECTION('',(0.,0.,1.));
#28520=DIRECTION('center_axis',(0.,0.,-1.));
#28521=DIRECTION('ref_axis',(-1.,0.,0.));
#28522=DIRECTION('center_axis',(0.,0.,-1.));
#28523=DIRECTION('ref_axis',(-1.,0.,0.));
#28524=DIRECTION('center_axis',(0.,0.,1.));
#28525=DIRECTION('ref_axis',(1.,0.,0.));
#28526=DIRECTION('',(1.,0.,0.));
#28527=DIRECTION('center_axis',(0.,0.,1.));
#28528=DIRECTION('ref_axis',(-0.707106781186547,-0.707106781186548,0.));
#28529=DIRECTION('',(0.,-1.,0.));
#28530=DIRECTION('center_axis',(0.,0.,1.));
#28531=DIRECTION('ref_axis',(-0.707106781186548,0.707106781186547,0.));
#28532=DIRECTION('',(-1.,0.,0.));
#28533=DIRECTION('',(0.,-1.,0.));
#28534=DIRECTION('center_axis',(0.,0.,1.));
#28535=DIRECTION('ref_axis',(-1.,0.,0.));
#28536=DIRECTION('center_axis',(0.,0.,1.));
#28537=DIRECTION('ref_axis',(-1.,0.,0.));
#28538=DIRECTION('',(-0.70710678118655,-8.65956056235496E-17,-0.707106781186545));
#28539=DIRECTION('center_axis',(0.,0.,1.));
#28540=DIRECTION('ref_axis',(1.,0.,0.));
#28541=DIRECTION('center_axis',(0.,0.,-1.));
#28542=DIRECTION('ref_axis',(0.707106781186549,-0.707106781186546,0.));
#28543=DIRECTION('',(0.,-1.,0.));
#28544=DIRECTION('center_axis',(0.,0.,-1.));
#28545=DIRECTION('ref_axis',(0.707106781186546,0.707106781186549,0.));
#28546=DIRECTION('',(1.,0.,0.));
#28547=DIRECTION('center_axis',(0.,0.,-1.));
#28548=DIRECTION('ref_axis',(-0.707106781186548,0.707106781186547,0.));
#28549=DIRECTION('',(0.,1.,0.));
#28550=DIRECTION('center_axis',(0.,0.,-1.));
#28551=DIRECTION('ref_axis',(-0.707106781186547,-0.707106781186548,0.));
#28552=DIRECTION('',(-1.,0.,0.));
#28553=DIRECTION('center_axis',(0.,0.707106781186547,-0.707106781186548));
#28554=DIRECTION('ref_axis',(-1.,0.,0.));
#28555=DIRECTION('',(0.,0.707106781186548,0.707106781186547));
#28556=DIRECTION('',(0.,0.707106781186548,0.707106781186547));
#28557=DIRECTION('',(1.,0.,0.));
#28558=DIRECTION('center_axis',(0.,0.,1.));
#28559=DIRECTION('ref_axis',(-0.707106781186548,0.707106781186547,0.));
#28560=DIRECTION('',(-0.70710678118654,0.,0.707106781186555));
#28561=DIRECTION('center_axis',(0.,0.,-1.));
#28562=DIRECTION('ref_axis',(-0.707106781186548,0.707106781186547,0.));
#28563=DIRECTION('center_axis',(-0.707106781186545,0.,-0.70710678118655));
#28564=DIRECTION('ref_axis',(-0.70710678118655,0.,0.707106781186545));
#28565=DIRECTION('',(-0.70710678118655,0.,0.707106781186545));
#28566=DIRECTION('',(0.,1.,0.));
#28567=DIRECTION('center_axis',(0.,0.,1.));
#28568=DIRECTION('ref_axis',(-0.707106781186547,-0.707106781186548,0.));
#28569=DIRECTION('',(0.,-0.707106781186546,0.707106781186549));
#28570=DIRECTION('center_axis',(0.,0.,-1.));
#28571=DIRECTION('ref_axis',(-0.707106781186547,-0.707106781186548,0.));
#28572=DIRECTION('center_axis',(0.,-0.707106781186547,-0.707106781186548));
#28573=DIRECTION('ref_axis',(-1.,0.,0.));
#28574=DIRECTION('',(0.,0.707106781186548,-0.707106781186547));
#28575=DIRECTION('',(-1.,0.,0.));
#28576=DIRECTION('center_axis',(-0.707106781186545,0.,-0.70710678118655));
#28577=DIRECTION('ref_axis',(-0.70710678118655,0.,0.707106781186545));
#28578=DIRECTION('',(0.,1.,0.));
#28579=DIRECTION('',(0.577350269189629,-0.577350269189625,-0.577350269189624));
#28580=DIRECTION('',(0.,-1.,0.));
#28581=DIRECTION('',(-0.577350269189629,-0.577350269189625,0.577350269189624));
#28582=DIRECTION('center_axis',(0.,-0.707106781186547,-0.707106781186548));
#28583=DIRECTION('ref_axis',(-1.,0.,0.));
#28584=DIRECTION('',(1.,0.,0.));
#28585=DIRECTION('',(0.,-0.707106781186548,0.707106781186547));
#28586=DIRECTION('',(-1.,0.,0.));
#28587=DIRECTION('center_axis',(0.,0.,1.));
#28588=DIRECTION('ref_axis',(0.707106781186549,-0.707106781186546,0.));
#28589=DIRECTION('',(0.707106781186561,0.,0.707106781186534));
#28590=DIRECTION('center_axis',(0.,0.,-1.));
#28591=DIRECTION('ref_axis',(0.707106781186549,-0.707106781186546,0.));
#28592=DIRECTION('center_axis',(0.,0.,1.));
#28593=DIRECTION('ref_axis',(0.707106781186549,-0.707106781186546,0.));
#28594=DIRECTION('center_axis',(0.707106781186545,0.,-0.70710678118655));
#28595=DIRECTION('ref_axis',(-0.70710678118655,0.,-0.707106781186545));
#28596=DIRECTION('',(0.70710678118655,6.54205191118237E-16,0.707106781186545));
#28597=DIRECTION('',(0.,-1.,0.));
#28598=DIRECTION('',(0.,1.,0.));
#28599=DIRECTION('center_axis',(0.,0.,1.));
#28600=DIRECTION('ref_axis',(0.707106781186546,0.707106781186549,0.));
#28601=DIRECTION('',(0.,0.707106781186552,0.707106781186543));
#28602=DIRECTION('center_axis',(0.,0.,-1.));
#28603=DIRECTION('ref_axis',(0.707106781186546,0.707106781186549,0.));
#28604=DIRECTION('center_axis',(0.,0.,1.));
#28605=DIRECTION('ref_axis',(0.707106781186546,0.707106781186549,0.));
#28606=DIRECTION('center_axis',(0.,0.707106781186547,-0.707106781186548));
#28607=DIRECTION('ref_axis',(-1.,0.,0.));
#28608=DIRECTION('',(1.,0.,0.));
#28609=DIRECTION('',(-1.,0.,0.));
#28610=DIRECTION('center_axis',(0.,0.,1.));
#28611=DIRECTION('ref_axis',(0.707106781186546,0.707106781186549,0.));
#28612=DIRECTION('',(0.,0.,1.));
#28613=DIRECTION('center_axis',(0.,0.,1.));
#28614=DIRECTION('ref_axis',(0.707106781186546,0.707106781186549,0.));
#28615=DIRECTION('',(0.,0.,-1.));
#28616=DIRECTION('center_axis',(0.,1.,0.));
#28617=DIRECTION('ref_axis',(-1.,0.,0.));
#28618=DIRECTION('',(0.,0.,-1.));
#28619=DIRECTION('',(-1.,0.,0.));
#28620=DIRECTION('',(0.,0.,1.));
#28621=DIRECTION('center_axis',(-1.,0.,0.));
#28622=DIRECTION('ref_axis',(0.,-1.,0.));
#28623=DIRECTION('',(0.,0.,1.));
#28624=DIRECTION('center_axis',(0.,0.,1.));
#28625=DIRECTION('ref_axis',(1.,0.,0.));
#28626=DIRECTION('center_axis',(0.,0.,-1.));
#28627=DIRECTION('ref_axis',(0.707106781186549,-0.707106781186546,0.));
#28628=DIRECTION('',(0.,-0.70710678118655,-0.707106781186545));
#28629=DIRECTION('center_axis',(0.,0.,1.));
#28630=DIRECTION('ref_axis',(0.707106781186549,-0.707106781186546,0.));
#28631=DIRECTION('',(-0.707106781186561,0.,0.707106781186534));
#28632=DIRECTION('center_axis',(0.,-0.707106781186548,0.707106781186548));
#28633=DIRECTION('ref_axis',(1.,0.,0.));
#28634=DIRECTION('',(0.,-0.707106781186548,-0.707106781186548));
#28635=DIRECTION('',(1.,0.,0.));
#28636=DIRECTION('center_axis',(0.,0.,-1.));
#28637=DIRECTION('ref_axis',(-0.707106781186547,-0.707106781186548,0.));
#28638=DIRECTION('',(-0.70710678118654,0.,-0.707106781186555));
#28639=DIRECTION('center_axis',(0.,0.,1.));
#28640=DIRECTION('ref_axis',(-0.707106781186547,-0.707106781186548,0.));
#28641=DIRECTION('center_axis',(-0.70710678118655,0.,0.707106781186545));
#28642=DIRECTION('ref_axis',(0.707106781186545,0.,0.70710678118655));
#28643=DIRECTION('',(-0.707106781186545,0.,-0.70710678118655));
#28644=DIRECTION('',(0.,-1.,0.));
#28645=DIRECTION('center_axis',(0.,0.,-1.));
#28646=DIRECTION('ref_axis',(-0.707106781186548,0.707106781186547,0.));
#28647=DIRECTION('',(0.,0.707106781186544,-0.707106781186551));
#28648=DIRECTION('center_axis',(0.,0.,1.));
#28649=DIRECTION('ref_axis',(-0.707106781186548,0.707106781186547,0.));
#28650=DIRECTION('center_axis',(0.,0.707106781186548,0.707106781186548));
#28651=DIRECTION('ref_axis',(1.,0.,0.));
#28652=DIRECTION('',(0.,0.707106781186548,-0.707106781186548));
#28653=DIRECTION('center_axis',(0.,0.,-1.));
#28654=DIRECTION('ref_axis',(0.707106781186546,0.707106781186549,0.));
#28655=DIRECTION('',(0.70710678118655,6.54205191118237E-16,-0.707106781186545));
#28656=DIRECTION('center_axis',(0.707106781186545,0.,0.70710678118655));
#28657=DIRECTION('ref_axis',(0.70710678118655,0.,-0.707106781186545));
#28658=DIRECTION('',(0.,1.,0.));
#28659=DIRECTION('center_axis',(1.,0.,0.));
#28660=DIRECTION('ref_axis',(0.,1.,0.));
#28661=DIRECTION('',(0.,0.,1.));
#28662=DIRECTION('center_axis',(0.,0.,1.));
#28663=DIRECTION('ref_axis',(0.707106781186549,-0.707106781186546,0.));
#28664=DIRECTION('',(0.,0.,-1.));
#28665=DIRECTION('center_axis',(0.,-1.,0.));
#28666=DIRECTION('ref_axis',(1.,0.,0.));
#28667=DIRECTION('',(0.,0.,1.));
#28668=DIRECTION('center_axis',(0.,0.,1.));
#28669=DIRECTION('ref_axis',(-0.707106781186547,-0.707106781186548,0.));
#28670=DIRECTION('',(0.,0.,-1.));
#28671=DIRECTION('center_axis',(-1.,0.,0.));
#28672=DIRECTION('ref_axis',(0.,-1.,0.));
#28673=DIRECTION('',(0.,0.,1.));
#28674=DIRECTION('center_axis',(0.,0.,1.));
#28675=DIRECTION('ref_axis',(-0.707106781186548,0.707106781186547,0.));
#35982=CARTESIAN_POINT('',(0.,0.,0.));
#35983=CARTESIAN_POINT('Origin',(4.6,0.,0.115));
#35984=CARTESIAN_POINT('',(4.345,3.12284933782576E-17,0.1));
#35985=CARTESIAN_POINT('Origin',(4.6,0.,0.1));
#35986=CARTESIAN_POINT('',(4.375,-2.75545529808155E-17,0.13));
#35987=CARTESIAN_POINT('',(4.36,2.93915231795366E-17,0.115));
#35988=CARTESIAN_POINT('Origin',(4.6,0.,0.13));
#35989=CARTESIAN_POINT('Origin',(4.6,0.,0.17));
#35990=CARTESIAN_POINT('',(4.375,-2.75545529808155E-17,0.27));
#35991=CARTESIAN_POINT('',(4.375,-2.75545529808155E-17,0.17));
#35992=CARTESIAN_POINT('',(4.825,-2.75545529808155E-17,0.27));
#35993=CARTESIAN_POINT('Origin',(4.6,0.,0.27));
#35994=CARTESIAN_POINT('Origin',(4.6,0.,0.27));
#35995=CARTESIAN_POINT('Origin',(4.55,0.,0.1));
#35996=CARTESIAN_POINT('',(3.8,-0.37,0.1));
#35997=CARTESIAN_POINT('',(5.25,-0.37,0.1));
#35998=CARTESIAN_POINT('',(4.,-0.37,0.1));
#35999=CARTESIAN_POINT('',(3.48,-0.05,0.1));
#36000=CARTESIAN_POINT('Origin',(3.8,-0.05,0.1));
#36001=CARTESIAN_POINT('',(3.48,0.05,0.1));
#36002=CARTESIAN_POINT('',(3.48,0.2,0.1));
#36003=CARTESIAN_POINT('',(3.8,0.37,0.1));
#36004=CARTESIAN_POINT('Origin',(3.8,0.05,0.1));
#36005=CARTESIAN_POINT('',(5.25,0.37,0.1));
#36006=CARTESIAN_POINT('',(5.1,0.37,0.1));
#36007=CARTESIAN_POINT('',(5.25,0.2,0.1));
#36008=CARTESIAN_POINT('Origin',(4.6,0.,0.285));
#36009=CARTESIAN_POINT('',(4.855,3.12284933782576E-17,0.3));
#36010=CARTESIAN_POINT('Origin',(4.6,0.,0.3));
#36011=CARTESIAN_POINT('',(4.84,2.93915231795366E-17,0.285));
#36012=CARTESIAN_POINT('Origin',(4.55,0.,0.3));
#36013=CARTESIAN_POINT('',(5.62,-0.2,0.3));
#36014=CARTESIAN_POINT('',(5.45,-0.37,0.3));
#36015=CARTESIAN_POINT('Origin',(5.45,-0.2,0.3));
#36016=CARTESIAN_POINT('',(5.62,0.2,0.3));
#36017=CARTESIAN_POINT('',(5.62,-0.2,0.3));
#36018=CARTESIAN_POINT('',(5.45,0.37,0.3));
#36019=CARTESIAN_POINT('Origin',(5.45,0.2,0.3));
#36020=CARTESIAN_POINT('',(3.8,0.37,0.3));
#36021=CARTESIAN_POINT('',(5.1,0.37,0.3));
#36022=CARTESIAN_POINT('',(3.48,0.05,0.3));
#36023=CARTESIAN_POINT('Origin',(3.8,0.05,0.3));
#36024=CARTESIAN_POINT('',(3.48,-0.05,0.3));
#36025=CARTESIAN_POINT('',(3.48,0.2,0.3));
#36026=CARTESIAN_POINT('',(3.8,-0.37,0.3));
#36027=CARTESIAN_POINT('Origin',(3.8,-0.05,0.3));
#36028=CARTESIAN_POINT('',(4.,-0.37,0.3));
#36029=CARTESIAN_POINT('Origin',(5.1,0.385,0.115));
#36030=CARTESIAN_POINT('',(5.25,0.4,0.13));
#36031=CARTESIAN_POINT('',(5.25,0.36,0.09));
#36032=CARTESIAN_POINT('',(3.8,0.4,0.13));
#36033=CARTESIAN_POINT('',(3.8,0.37,0.1));
#36034=CARTESIAN_POINT('',(5.1,0.4,0.13));
#36035=CARTESIAN_POINT('Origin',(3.8,0.05,0.115));
#36036=CARTESIAN_POINT('',(3.45,0.05,0.13));
#36037=CARTESIAN_POINT('',(3.48,0.05,0.1));
#36038=CARTESIAN_POINT('Origin',(3.8,0.05,0.13));
#36039=CARTESIAN_POINT('Origin',(3.465,0.2,0.115));
#36040=CARTESIAN_POINT('',(3.45,-0.05,0.13));
#36041=CARTESIAN_POINT('',(3.48,-0.05,0.1));
#36042=CARTESIAN_POINT('',(3.45,0.2,0.13));
#36043=CARTESIAN_POINT('Origin',(3.8,-0.05,0.115));
#36044=CARTESIAN_POINT('',(3.8,-0.4,0.13));
#36045=CARTESIAN_POINT('',(3.8,-0.37,0.1));
#36046=CARTESIAN_POINT('Origin',(3.8,-0.05,0.13));
#36047=CARTESIAN_POINT('Origin',(4.,-0.385,0.115));
#36048=CARTESIAN_POINT('',(5.25,-0.4,0.13));
#36049=CARTESIAN_POINT('',(5.25,-0.16,-0.11));
#36050=CARTESIAN_POINT('',(4.,-0.4,0.13));
#36051=CARTESIAN_POINT('Origin',(5.265,0.2,0.015));
#36052=CARTESIAN_POINT('',(5.25,-0.4,0.03));
#36053=CARTESIAN_POINT('',(5.25,0.4,0.03));
#36054=CARTESIAN_POINT('',(5.25,0.2,0.03));
#36055=CARTESIAN_POINT('',(5.28,0.37,0.));
#36056=CARTESIAN_POINT('',(5.25,0.4,0.03));
#36057=CARTESIAN_POINT('',(5.28,-0.37,0.));
#36058=CARTESIAN_POINT('',(5.28,0.2,0.));
#36059=CARTESIAN_POINT('',(5.28,-0.37,0.));
#36060=CARTESIAN_POINT('Origin',(4.45,-0.385,0.015));
#36061=CARTESIAN_POINT('',(5.45,-0.37,0.));
#36062=CARTESIAN_POINT('',(4.45,-0.37,0.));
#36063=CARTESIAN_POINT('',(5.45,-0.4,0.03));
#36064=CARTESIAN_POINT('',(5.45,-0.37,0.));
#36065=CARTESIAN_POINT('',(4.45,-0.4,0.03));
#36066=CARTESIAN_POINT('Origin',(5.45,-0.2,0.015));
#36067=CARTESIAN_POINT('',(5.62,-0.2,0.));
#36068=CARTESIAN_POINT('',(5.65,-0.2,0.03));
#36069=CARTESIAN_POINT('',(5.62,-0.2,0.));
#36070=CARTESIAN_POINT('Origin',(5.45,-0.2,0.03));
#36071=CARTESIAN_POINT('Origin',(5.45,-0.2,0.));
#36072=CARTESIAN_POINT('Origin',(5.635,-0.2,0.015));
#36073=CARTESIAN_POINT('',(5.62,0.2,0.));
#36074=CARTESIAN_POINT('',(5.65,0.2,0.03));
#36075=CARTESIAN_POINT('',(5.62,0.2,0.));
#36076=CARTESIAN_POINT('',(5.65,-0.2,0.03));
#36077=CARTESIAN_POINT('',(5.62,-0.2,0.));
#36078=CARTESIAN_POINT('Origin',(5.45,0.2,0.015));
#36079=CARTESIAN_POINT('',(5.45,0.37,0.));
#36080=CARTESIAN_POINT('',(5.45,0.4,0.03));
#36081=CARTESIAN_POINT('',(5.45,0.37,0.));
#36082=CARTESIAN_POINT('Origin',(5.45,0.2,0.03));
#36083=CARTESIAN_POINT('Origin',(5.45,0.2,0.));
#36084=CARTESIAN_POINT('Origin',(5.55,0.385,0.015));
#36085=CARTESIAN_POINT('',(5.55,0.4,0.03));
#36086=CARTESIAN_POINT('',(5.55,0.37,0.));
#36087=CARTESIAN_POINT('Origin',(5.45,0.2,0.1));
#36088=CARTESIAN_POINT('',(5.45,0.4,0.27));
#36089=CARTESIAN_POINT('',(5.45,0.4,0.1));
#36090=CARTESIAN_POINT('',(5.65,0.2,0.27));
#36091=CARTESIAN_POINT('Origin',(5.45,0.2,0.27));
#36092=CARTESIAN_POINT('',(5.65,0.2,0.1));
#36093=CARTESIAN_POINT('Origin',(5.65,0.4,0.1));
#36094=CARTESIAN_POINT('',(3.8,0.4,0.27));
#36095=CARTESIAN_POINT('',(3.8,0.4,0.1));
#36096=CARTESIAN_POINT('',(5.1,0.4,0.27));
#36097=CARTESIAN_POINT('',(5.25,0.4,0.));
#36098=CARTESIAN_POINT('Origin',(5.25,0.4,0.));
#36099=CARTESIAN_POINT('',(5.25,-0.4,0.));
#36100=CARTESIAN_POINT('Origin',(5.45,0.,0.));
#36101=CARTESIAN_POINT('Origin',(5.45,-0.2,0.285));
#36102=CARTESIAN_POINT('',(5.45,-0.4,0.27));
#36103=CARTESIAN_POINT('',(5.45,-0.37,0.3));
#36104=CARTESIAN_POINT('',(5.65,-0.2,0.27));
#36105=CARTESIAN_POINT('Origin',(5.45,-0.2,0.27));
#36106=CARTESIAN_POINT('',(5.65,-0.2,0.27));
#36107=CARTESIAN_POINT('Origin',(4.,-0.385,0.285));
#36108=CARTESIAN_POINT('',(3.8,-0.4,0.27));
#36109=CARTESIAN_POINT('',(3.8,-0.37,0.3));
#36110=CARTESIAN_POINT('',(4.,-0.4,0.27));
#36111=CARTESIAN_POINT('Origin',(3.8,-0.05,0.285));
#36112=CARTESIAN_POINT('',(3.45,-0.05,0.27));
#36113=CARTESIAN_POINT('',(3.48,-0.05,0.3));
#36114=CARTESIAN_POINT('Origin',(3.8,-0.05,0.27));
#36115=CARTESIAN_POINT('Origin',(3.465,0.2,0.285));
#36116=CARTESIAN_POINT('',(3.45,0.05,0.27));
#36117=CARTESIAN_POINT('',(3.48,0.05,0.3));
#36118=CARTESIAN_POINT('',(3.45,0.2,0.27));
#36119=CARTESIAN_POINT('Origin',(3.8,0.05,0.285));
#36120=CARTESIAN_POINT('',(3.8,0.37,0.3));
#36121=CARTESIAN_POINT('Origin',(3.8,0.05,0.27));
#36122=CARTESIAN_POINT('Origin',(5.1,0.385,0.285));
#36123=CARTESIAN_POINT('',(5.45,0.37,0.3));
#36124=CARTESIAN_POINT('Origin',(5.45,0.2,0.285));
#36125=CARTESIAN_POINT('',(5.62,0.2,0.3));
#36126=CARTESIAN_POINT('Origin',(5.635,-0.2,0.285));
#36127=CARTESIAN_POINT('',(5.65,-0.2,0.27));
#36128=CARTESIAN_POINT('Origin',(5.65,-0.4,0.1));
#36129=CARTESIAN_POINT('',(5.65,-0.2,0.1));
#36130=CARTESIAN_POINT('Origin',(5.45,-0.2,0.1));
#36131=CARTESIAN_POINT('',(5.45,-0.4,0.1));
#36132=CARTESIAN_POINT('Origin',(3.45,-0.4,0.1));
#36133=CARTESIAN_POINT('',(3.8,-0.4,0.1));
#36134=CARTESIAN_POINT('Origin',(3.8,-0.05,0.1));
#36135=CARTESIAN_POINT('',(3.45,-0.05,0.1));
#36136=CARTESIAN_POINT('Origin',(3.45,0.4,0.1));
#36137=CARTESIAN_POINT('',(3.45,0.05,0.1));
#36138=CARTESIAN_POINT('Origin',(3.8,0.05,0.1));
#53626=UNCERTAINTY_MEASURE_WITH_UNIT(LENGTH_MEASURE(0.001),#53651,
'DISTANCE_ACCURACY_VALUE',
'Maximum model space distance between geometric entities at asserted c
onnectivities');
#53632=UNCERTAINTY_MEASURE_WITH_UNIT(LENGTH_MEASURE(0.001),#53651,
'DISTANCE_ACCURACY_VALUE',
'Maximum model space distance between geometric entities at asserted c
onnectivities');
#53644=(
GEOMETRIC_REPRESENTATION_CONTEXT(3)
GLOBAL_UNCERTAINTY_ASSIGNED_CONTEXT((#53626))
GLOBAL_UNIT_ASSIGNED_CONTEXT((#53651,#53653,#53654))
REPRESENTATION_CONTEXT('','3D')
);
#53650=(
GEOMETRIC_REPRESENTATION_CONTEXT(3)
GLOBAL_UNCERTAINTY_ASSIGNED_CONTEXT((#53632))
GLOBAL_UNIT_ASSIGNED_CONTEXT((#53651,#53653,#53654))
REPRESENTATION_CONTEXT('','3D')
);
#53651=(
LENGTH_UNIT()
NAMED_UNIT(*)
SI_UNIT(.CENTI.,.METRE.)
);
#53653=(
NAMED_UNIT(*)
PLANE_ANGLE_UNIT()
SI_UNIT($,.RADIAN.)
);
#53654=(
NAMED_UNIT(*)
SI_UNIT($,.STERADIAN.)
SOLID_ANGLE_UNIT()
);
#53666=SHAPE_DEFINITION_REPRESENTATION(#53683,#53734);
#53683=PRODUCT_DEFINITION_SHAPE('',$,#53752);
#53734=SHAPE_REPRESENTATION('',(#24530),#53644);
#53740=PRODUCT_DEFINITION_CONTEXT('part definition',#53793,'design');
#53752=PRODUCT_DEFINITION('2026-10-18-22-44-43-794',
'09_Mirror_Retaining_Clip',#53769,#53740);
#53769=PRODUCT_DEFINITION_FORMATION('',$,#53806);
#53793=APPLICATION_CONTEXT(
'Core Data for Automotive Mechanical Design Process');
#53794=PRODUCT_CONTEXT('part definition',#53793,'mechanical');
#53806=PRODUCT('2026-10-18-22-44-43-794','09_Mirror_Retaining_Clip',$,(#53794));
#53945=COLOUR_RGB('Sky Blue',0.24,0.69,0.87);
#53946=FILL_AREA_STYLE_COLOUR('',#53945);
#53947=FILL_AREA_STYLE('',(#53946));
#53948=SURFACE_STYLE_FILL_AREA(#53947);
#53949=SURFACE_SIDE_STYLE('',(#53948));
#53950=SURFACE_STYLE_USAGE(.BOTH.,#53949);
#53951=PRESENTATION_STYLE_ASSIGNMENT((#53950));
ENDSEC;
END-ISO-10303-21;
